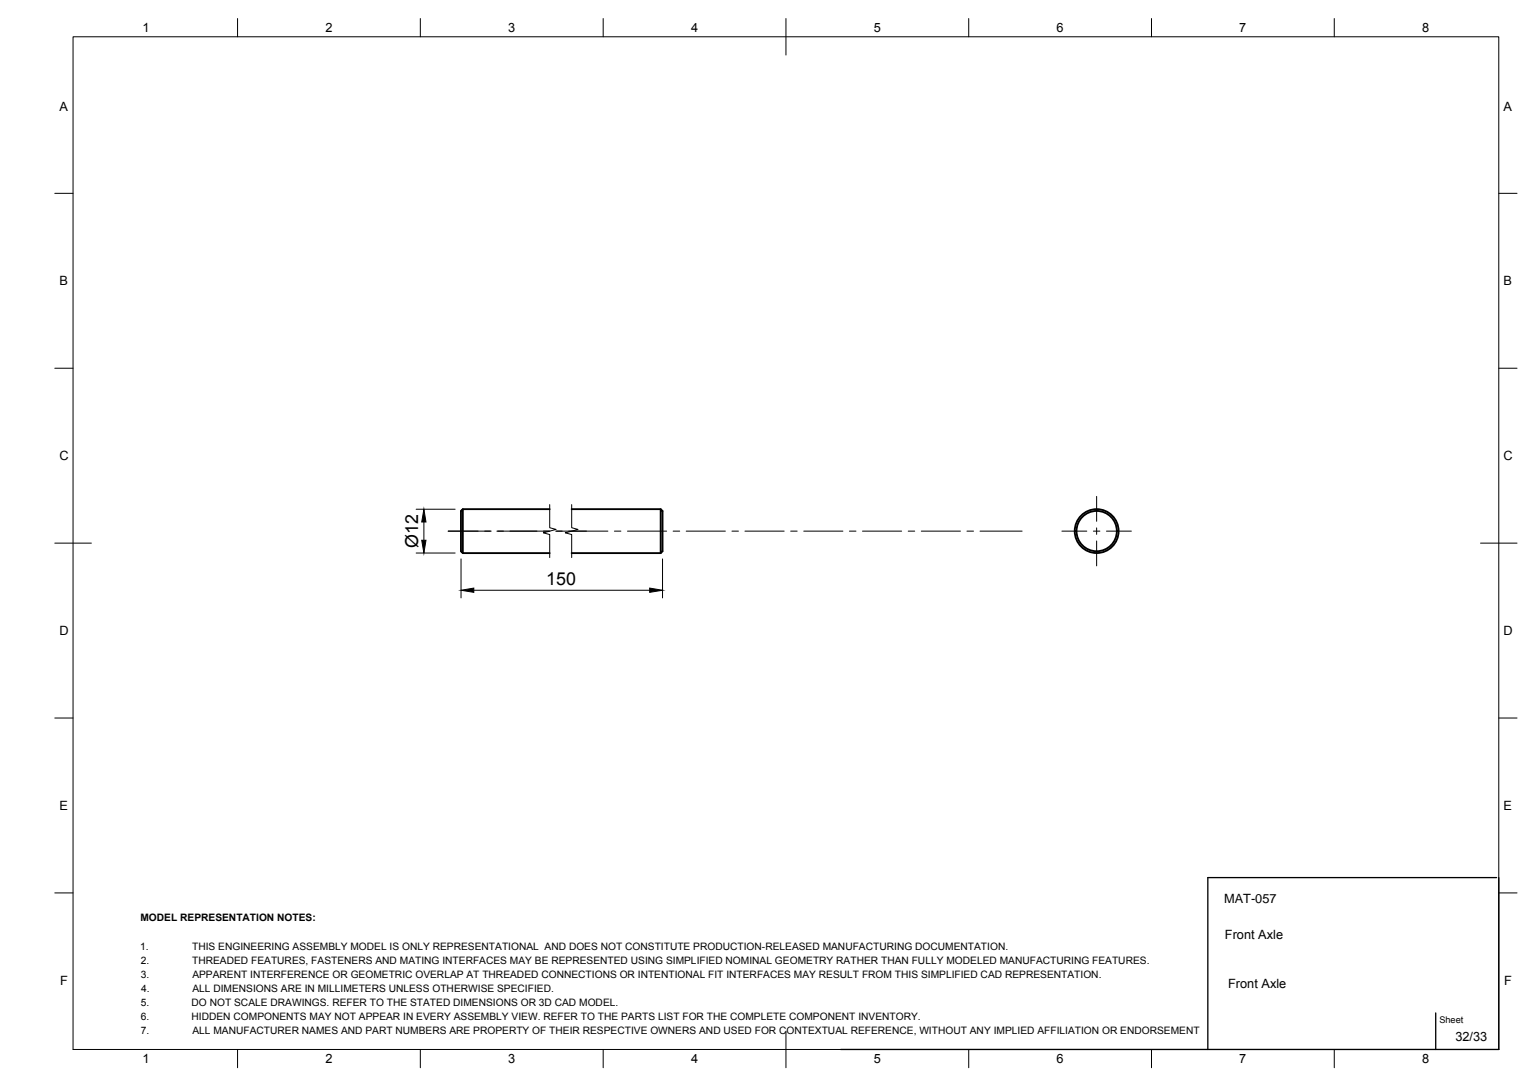
ISO-10303-21;
HEADER;
/* Generated by software containing ST-Developer
 * from STEP Tools, Inc. (www.steptools.com) 
 */

FILE_DESCRIPTION(
/* description */ ('STEP AP214', 'CAx-IF Rec.Pracs.---Representation and Presentation of Product Manufa
cturing Information (PMI)---4.0---2014-10-13'),
/* implementation_level */ '2;1');

FILE_NAME(
/* name */ 'Front Axle.step',
/* time_stamp */ '2026-10-28T23:34:22+01:00',
/* author */ (''),
/* organization */ (''),
/* preprocessor_version */ 'ST-DEVELOPER v20.2',
/* originating_system */ 'Autodesk Translation Framework v15.17.0.0',
/* authorisation */ '');

FILE_SCHEMA (('AP242_MANAGED_MODEL_BASED_3D_ENGINEERING_MIM_LF { 1 0 10303 442 2 1 4 }'));
ENDSEC;

DATA;
#10=MECHANICAL_DESIGN_GEOMETRIC_PRESENTATION_REPRESENTATION('',(#271),#27807);
#223=SHAPE_REPRESENTATION_RELATIONSHIP('SRR','None',#27922,#245);
#245=ADVANCED_BREP_SHAPE_REPRESENTATION('',(#300),#27802);
#271=STYLED_ITEM('',(#28077),#300);
#300=MANIFOLD_SOLID_BREP('Body1',#12047);
#693=PLANE('',#13465);
#694=PLANE('',#13466);
#1179=CYLINDRICAL_SURFACE('',#13464,6.);
#1793=FACE_OUTER_BOUND('',#2582,.T.);
#1794=FACE_OUTER_BOUND('',#2583,.T.);
#1795=FACE_OUTER_BOUND('',#2584,.T.);
#1796=FACE_OUTER_BOUND('',#2585,.T.);
#1797=FACE_OUTER_BOUND('',#2586,.T.);
#2582=EDGE_LOOP('',(#10563,#10564,#10565,#10566));
#2583=EDGE_LOOP('',(#10567,#10568,#10569,#10570,#10571));
#2584=EDGE_LOOP('',(#10572,#10573,#10574,#10575,#10576));
#2585=EDGE_LOOP('',(#10577));
#2586=EDGE_LOOP('',(#10578));
#3422=LINE('',#23220,#4242);
#3423=LINE('',#23228,#4243);
#3424=LINE('',#23231,#4244);
#4242=VECTOR('',#16722,5.49999999999999);
#4243=VECTOR('',#16731,6.);
#4244=VECTOR('',#16736,6.);
#4935=CIRCLE('',#13458,6.00000000000001);
#4936=CIRCLE('',#13459,5.49999999999999);
#4937=CIRCLE('',#13461,6.);
#4938=CIRCLE('',#13462,6.);
#4939=CIRCLE('',#13463,5.49999999999997);
#5905=VERTEX_POINT('',#23217);
#5906=VERTEX_POINT('',#23219);
#5907=VERTEX_POINT('',#23223);
#5908=VERTEX_POINT('',#23224);
#5909=VERTEX_POINT('',#23227);
#7494=EDGE_CURVE('',#5905,#5905,#4935,.T.);
#7495=EDGE_CURVE('',#5905,#5906,#3422,.T.);
#7496=EDGE_CURVE('',#5906,#5906,#4936,.T.);
#7497=EDGE_CURVE('',#5907,#5908,#4937,.T.);
#7498=EDGE_CURVE('',#5908,#5907,#4938,.T.);
#7499=EDGE_CURVE('',#5908,#5909,#3423,.T.);
#7500=EDGE_CURVE('',#5909,#5909,#4939,.T.);
#7501=EDGE_CURVE('',#5907,#5905,#3424,.T.);
#10563=ORIENTED_EDGE('',*,*,#7494,.F.);
#10564=ORIENTED_EDGE('',*,*,#7495,.T.);
#10565=ORIENTED_EDGE('',*,*,#7496,.F.);
#10566=ORIENTED_EDGE('',*,*,#7495,.F.);
#10567=ORIENTED_EDGE('',*,*,#7497,.F.);
#10568=ORIENTED_EDGE('',*,*,#7498,.F.);
#10569=ORIENTED_EDGE('',*,*,#7499,.T.);
#10570=ORIENTED_EDGE('',*,*,#7500,.F.);
#10571=ORIENTED_EDGE('',*,*,#7499,.F.);
#10572=ORIENTED_EDGE('',*,*,#7497,.T.);
#10573=ORIENTED_EDGE('',*,*,#7498,.T.);
#10574=ORIENTED_EDGE('',*,*,#7501,.T.);
#10575=ORIENTED_EDGE('',*,*,#7494,.T.);
#10576=ORIENTED_EDGE('',*,*,#7501,.F.);
#10577=ORIENTED_EDGE('',*,*,#7496,.T.);
#10578=ORIENTED_EDGE('',*,*,#7500,.T.);
#11312=CONICAL_SURFACE('',#13457,5.49999999999999,0.785398163397442);
#11313=CONICAL_SURFACE('',#13460,6.,0.785398163397442);
#11875=ADVANCED_FACE('',(#1793),#11312,.T.);
#11876=ADVANCED_FACE('',(#1794),#11313,.T.);
#11877=ADVANCED_FACE('',(#1795),#1179,.T.);
#11878=ADVANCED_FACE('',(#1796),#693,.T.);
#11879=ADVANCED_FACE('',(#1797),#694,.F.);
#12047=CLOSED_SHELL('',(#11875,#11876,#11877,#11878,#11879));
#13456=AXIS2_PLACEMENT_3D('',#23215,#16716,#16717);
#13457=AXIS2_PLACEMENT_3D('',#23216,#16718,#16719);
#13458=AXIS2_PLACEMENT_3D('',#23218,#16720,#16721);
#13459=AXIS2_PLACEMENT_3D('',#23221,#16723,#16724);
#13460=AXIS2_PLACEMENT_3D('',#23222,#16725,#16726);
#13461=AXIS2_PLACEMENT_3D('',#23225,#16727,#16728);
#13462=AXIS2_PLACEMENT_3D('',#23226,#16729,#16730);
#13463=AXIS2_PLACEMENT_3D('',#23229,#16732,#16733);
#13464=AXIS2_PLACEMENT_3D('',#23230,#16734,#16735);
#13465=AXIS2_PLACEMENT_3D('',#23232,#16737,#16738);
#13466=AXIS2_PLACEMENT_3D('',#23233,#16739,#16740);
#16716=DIRECTION('axis',(0.,0.,1.));
#16717=DIRECTION('refdir',(1.,0.,0.));
#16718=DIRECTION('center_axis',(0.,0.,-1.));
#16719=DIRECTION('ref_axis',(-0.537828840392936,-0.843054054282162,0.));
#16720=DIRECTION('center_axis',(0.,0.,-1.));
#16721=DIRECTION('ref_axis',(0.537828840392939,0.843054054282159,0.));
#16722=DIRECTION('',(-0.38030242015954,-0.596129238689725,0.707106781186552));
#16723=DIRECTION('center_axis',(0.,0.,1.));
#16724=DIRECTION('ref_axis',(0.537828840392936,0.843054054282162,0.));
#16725=DIRECTION('center_axis',(0.,0.,1.));
#16726=DIRECTION('ref_axis',(0.53782884039294,0.843054054282159,0.));
#16727=DIRECTION('center_axis',(0.,0.,1.));
#16728=DIRECTION('ref_axis',(0.53782884039294,0.843054054282159,0.));
#16729=DIRECTION('center_axis',(0.,0.,1.));
#16730=DIRECTION('ref_axis',(0.53782884039294,0.843054054282159,0.));
#16731=DIRECTION('',(0.380302420159543,0.596129238689723,-0.707106781186552));
#16732=DIRECTION('center_axis',(0.,0.,-1.));
#16733=DIRECTION('ref_axis',(0.537828840392938,0.84305405428216,0.));
#16734=DIRECTION('center_axis',(0.,0.,-1.));
#16735=DIRECTION('ref_axis',(-0.53782884039294,-0.843054054282159,0.));
#16736=DIRECTION('',(0.,0.,1.));
#16737=DIRECTION('center_axis',(0.,0.,1.));
#16738=DIRECTION('ref_axis',(0.537828840392939,0.84305405428216,0.));
#16739=DIRECTION('center_axis',(0.,0.,1.));
#16740=DIRECTION('ref_axis',(0.537828840392939,0.84305405428216,0.));
#23215=CARTESIAN_POINT('',(0.,0.,0.));
#23216=CARTESIAN_POINT('Origin',(-276.958747352154,52.7397376070391,327.735519388031));
#23217=CARTESIAN_POINT('',(-273.731774309796,57.7980619327321,327.235519388031));
#23218=CARTESIAN_POINT('Origin',(-276.958747352154,52.7397376070391,327.235519388031));
#23219=CARTESIAN_POINT('',(-274.000688729993,57.376534905591,327.735519388031));
#23220=CARTESIAN_POINT('',(-274.000688729993,57.376534905591,327.735519388031));
#23221=CARTESIAN_POINT('Origin',(-276.958747352154,52.7397376070391,327.735519388031));
#23222=CARTESIAN_POINT('Origin',(-276.958747352154,52.7397376070391,178.235519388031));
#23223=CARTESIAN_POINT('',(-273.731774309796,57.7980619327321,178.235519388031));
#23224=CARTESIAN_POINT('',(-280.185720394511,47.6814132813461,178.235519388031));
#23225=CARTESIAN_POINT('Origin',(-276.958747352154,52.7397376070391,178.235519388031));
#23226=CARTESIAN_POINT('Origin',(-276.958747352154,52.7397376070391,178.235519388031));
#23227=CARTESIAN_POINT('',(-279.916805974315,48.1029403084872,177.735519388031));
#23228=CARTESIAN_POINT('',(-280.185720394511,47.6814132813461,178.235519388031));
#23229=CARTESIAN_POINT('Origin',(-276.958747352154,52.7397376070391,177.735519388031));
#23230=CARTESIAN_POINT('Origin',(-276.958747352154,52.7397376070391,327.735519388031));
#23231=CARTESIAN_POINT('',(-273.731774309796,57.7980619327321,327.735519388031));
#23232=CARTESIAN_POINT('Origin',(-276.958747352154,52.7397376070391,327.735519388031));
#23233=CARTESIAN_POINT('Origin',(-276.958747352154,52.7397376070391,177.735519388031));
#27773=UNCERTAINTY_MEASURE_WITH_UNIT(LENGTH_MEASURE(0.01),#27808,
'DISTANCE_ACCURACY_VALUE',
'Maximum model space distance between geometric entities at asserted c
onnectivities');
#27778=UNCERTAINTY_MEASURE_WITH_UNIT(LENGTH_MEASURE(0.01),#27808,
'DISTANCE_ACCURACY_VALUE',
'Maximum model space distance between geometric entities at asserted c
onnectivities');
#27802=(
GEOMETRIC_REPRESENTATION_CONTEXT(3)
GLOBAL_UNCERTAINTY_ASSIGNED_CONTEXT((#27773))
GLOBAL_UNIT_ASSIGNED_CONTEXT((#27808,#27810,#27811))
REPRESENTATION_CONTEXT('','3D')
);
#27807=(
GEOMETRIC_REPRESENTATION_CONTEXT(3)
GLOBAL_UNCERTAINTY_ASSIGNED_CONTEXT((#27778))
GLOBAL_UNIT_ASSIGNED_CONTEXT((#27808,#27810,#27811))
REPRESENTATION_CONTEXT('','3D')
);
#27808=(
LENGTH_UNIT()
NAMED_UNIT(*)
SI_UNIT(.MILLI.,.METRE.)
);
#27810=(
NAMED_UNIT(*)
PLANE_ANGLE_UNIT()
SI_UNIT($,.RADIAN.)
);
#27811=(
NAMED_UNIT(*)
SI_UNIT($,.STERADIAN.)
SOLID_ANGLE_UNIT()
);
#27835=SHAPE_DEFINITION_REPRESENTATION(#27878,#27922);
#27878=PRODUCT_DEFINITION_SHAPE('',$,#27951);
#27922=SHAPE_REPRESENTATION('',(#13456),#27802);
#27927=PRODUCT_DEFINITION_CONTEXT('part definition',#28013,'design');
#27951=PRODUCT_DEFINITION('Front Axle','Front Axle',#27979,#27927);
#27979=PRODUCT_DEFINITION_FORMATION('',$,#28038);
#28013=APPLICATION_CONTEXT('Managed model based 3d engineering');
#28014=PRODUCT_CONTEXT('part definition',#28013,'mechanical');
#28038=PRODUCT('Front Axle','Front Axle',$,(#28014));
#28071=COLOUR_RGB('Grey',0.48,0.52,0.57);
#28072=FILL_AREA_STYLE_COLOUR('',#28071);
#28073=FILL_AREA_STYLE('',(#28072));
#28074=SURFACE_STYLE_FILL_AREA(#28073);
#28075=SURFACE_SIDE_STYLE('',(#28074));
#28076=SURFACE_STYLE_USAGE(.BOTH.,#28075);
#28077=PRESENTATION_STYLE_ASSIGNMENT((#28076));
ENDSEC;
END-ISO-10303-21;
